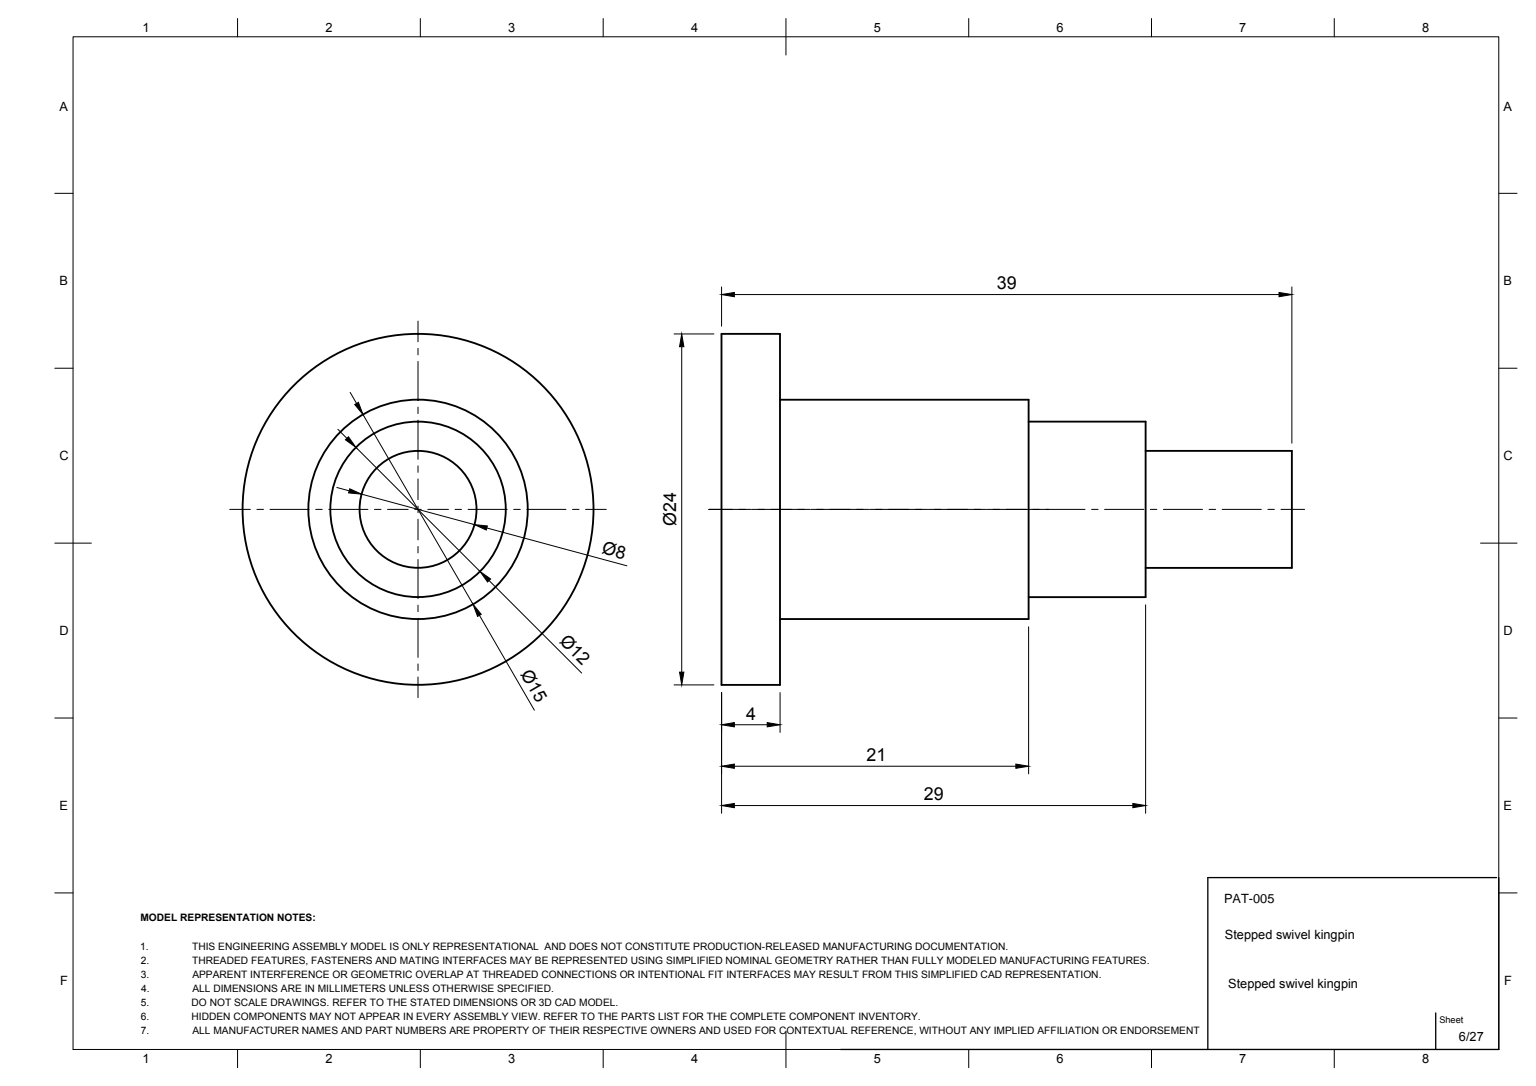
ISO-10303-21;
HEADER;
/* Generated by software containing ST-Developer
 * from STEP Tools, Inc. (www.steptools.com) 
 */

FILE_DESCRIPTION(
/* description */ ('Ball-race swivel caster'),
/* implementation_level */ '2;1');

FILE_NAME(
/* name */ 'Stepped swivel kingpin.step',
/* time_stamp */ '2026-10-29T16:15:51-07:00',
/* author */ (''),
/* organization */ (''),
/* preprocessor_version */ 'ST-DEVELOPER v20.2',
/* originating_system */ 'Autodesk Translation Framework v15.17.0.0',
/* authorisation */ '');

FILE_SCHEMA (('AUTOMOTIVE_DESIGN { 1 0 10303 214 3 1 1 }'));
ENDSEC;

DATA;
#10=MECHANICAL_DESIGN_GEOMETRIC_PRESENTATION_REPRESENTATION('',(#299),#7816);
#259=SHAPE_REPRESENTATION_RELATIONSHIP('SRR','None',#7904,#279);
#279=ADVANCED_BREP_SHAPE_REPRESENTATION('',(#335),#7793);
#299=STYLED_ITEM('',(#8097),#335);
#335=MANIFOLD_SOLID_BREP('Body1',#3705);
#379=FACE_BOUND('',#757,.T.);
#380=FACE_BOUND('',#761,.T.);
#381=FACE_BOUND('',#765,.T.);
#444=PLANE('',#3990);
#445=PLANE('',#3991);
#446=PLANE('',#3996);
#447=PLANE('',#3997);
#448=PLANE('',#4003);
#535=FACE_OUTER_BOUND('',#754,.T.);
#536=FACE_OUTER_BOUND('',#755,.T.);
#537=FACE_OUTER_BOUND('',#756,.T.);
#538=FACE_OUTER_BOUND('',#758,.T.);
#539=FACE_OUTER_BOUND('',#759,.T.);
#540=FACE_OUTER_BOUND('',#760,.T.);
#541=FACE_OUTER_BOUND('',#762,.T.);
#542=FACE_OUTER_BOUND('',#763,.T.);
#543=FACE_OUTER_BOUND('',#764,.T.);
#754=EDGE_LOOP('',(#2487,#2488,#2489,#2490));
#755=EDGE_LOOP('',(#2491));
#756=EDGE_LOOP('',(#2492));
#757=EDGE_LOOP('',(#2493));
#758=EDGE_LOOP('',(#2494,#2495,#2496,#2497));
#759=EDGE_LOOP('',(#2498));
#760=EDGE_LOOP('',(#2499));
#761=EDGE_LOOP('',(#2500));
#762=EDGE_LOOP('',(#2501,#2502,#2503,#2504));
#763=EDGE_LOOP('',(#2505,#2506,#2507,#2508));
#764=EDGE_LOOP('',(#2509));
#765=EDGE_LOOP('',(#2510));
#1028=LINE('',#5762,#1183);
#1029=LINE('',#5773,#1184);
#1030=LINE('',#5781,#1185);
#1031=LINE('',#5784,#1186);
#1183=VECTOR('',#4560,0.4);
#1184=VECTOR('',#4575,1.2);
#1185=VECTOR('',#4586,0.75);
#1186=VECTOR('',#4589,0.6);
#1331=CIRCLE('',#3988,0.4);
#1332=CIRCLE('',#3989,0.4);
#1333=CIRCLE('',#3992,1.2);
#1334=CIRCLE('',#3993,0.75);
#1335=CIRCLE('',#3995,1.2);
#1336=CIRCLE('',#3998,0.75);
#1337=CIRCLE('',#3999,0.6);
#1338=CIRCLE('',#4002,0.6);
#1603=VERTEX_POINT('',#5759);
#1604=VERTEX_POINT('',#5761);
#1605=VERTEX_POINT('',#5766);
#1606=VERTEX_POINT('',#5768);
#1607=VERTEX_POINT('',#5771);
#1608=VERTEX_POINT('',#5776);
#1609=VERTEX_POINT('',#5778);
#1610=VERTEX_POINT('',#5783);
#1963=EDGE_CURVE('',#1603,#1603,#1331,.T.);
#1964=EDGE_CURVE('',#1603,#1604,#1028,.T.);
#1965=EDGE_CURVE('',#1604,#1604,#1332,.T.);
#1966=EDGE_CURVE('',#1605,#1605,#1333,.T.);
#1967=EDGE_CURVE('',#1606,#1606,#1334,.T.);
#1968=EDGE_CURVE('',#1607,#1607,#1335,.T.);
#1969=EDGE_CURVE('',#1607,#1605,#1029,.T.);
#1970=EDGE_CURVE('',#1608,#1608,#1336,.T.);
#1971=EDGE_CURVE('',#1609,#1609,#1337,.T.);
#1972=EDGE_CURVE('',#1606,#1608,#1030,.T.);
#1973=EDGE_CURVE('',#1609,#1610,#1031,.T.);
#1974=EDGE_CURVE('',#1610,#1610,#1338,.T.);
#2487=ORIENTED_EDGE('',*,*,#1963,.F.);
#2488=ORIENTED_EDGE('',*,*,#1964,.T.);
#2489=ORIENTED_EDGE('',*,*,#1965,.T.);
#2490=ORIENTED_EDGE('',*,*,#1964,.F.);
#2491=ORIENTED_EDGE('',*,*,#1965,.F.);
#2492=ORIENTED_EDGE('',*,*,#1966,.F.);
#2493=ORIENTED_EDGE('',*,*,#1967,.T.);
#2494=ORIENTED_EDGE('',*,*,#1968,.F.);
#2495=ORIENTED_EDGE('',*,*,#1969,.T.);
#2496=ORIENTED_EDGE('',*,*,#1966,.T.);
#2497=ORIENTED_EDGE('',*,*,#1969,.F.);
#2498=ORIENTED_EDGE('',*,*,#1968,.T.);
#2499=ORIENTED_EDGE('',*,*,#1970,.F.);
#2500=ORIENTED_EDGE('',*,*,#1971,.T.);
#2501=ORIENTED_EDGE('',*,*,#1967,.F.);
#2502=ORIENTED_EDGE('',*,*,#1972,.T.);
#2503=ORIENTED_EDGE('',*,*,#1970,.T.);
#2504=ORIENTED_EDGE('',*,*,#1972,.F.);
#2505=ORIENTED_EDGE('',*,*,#1971,.F.);
#2506=ORIENTED_EDGE('',*,*,#1973,.T.);
#2507=ORIENTED_EDGE('',*,*,#1974,.T.);
#2508=ORIENTED_EDGE('',*,*,#1973,.F.);
#2509=ORIENTED_EDGE('',*,*,#1974,.F.);
#2510=ORIENTED_EDGE('',*,*,#1963,.T.);
#3432=CYLINDRICAL_SURFACE('',#3987,0.4);
#3433=CYLINDRICAL_SURFACE('',#3994,1.2);
#3434=CYLINDRICAL_SURFACE('',#4000,0.75);
#3435=CYLINDRICAL_SURFACE('',#4001,0.6);
#3506=ADVANCED_FACE('',(#535),#3432,.T.);
#3507=ADVANCED_FACE('',(#536),#444,.F.);
#3508=ADVANCED_FACE('',(#537,#379),#445,.F.);
#3509=ADVANCED_FACE('',(#538),#3433,.T.);
#3510=ADVANCED_FACE('',(#539),#446,.T.);
#3511=ADVANCED_FACE('',(#540,#380),#447,.F.);
#3512=ADVANCED_FACE('',(#541),#3434,.T.);
#3513=ADVANCED_FACE('',(#542),#3435,.T.);
#3514=ADVANCED_FACE('',(#543,#381),#448,.F.);
#3705=CLOSED_SHELL('',(#3506,#3507,#3508,#3509,#3510,#3511,#3512,#3513,
#3514));
#3986=AXIS2_PLACEMENT_3D('',#5757,#4554,#4555);
#3987=AXIS2_PLACEMENT_3D('',#5758,#4556,#4557);
#3988=AXIS2_PLACEMENT_3D('',#5760,#4558,#4559);
#3989=AXIS2_PLACEMENT_3D('',#5763,#4561,#4562);
#3990=AXIS2_PLACEMENT_3D('',#5764,#4563,#4564);
#3991=AXIS2_PLACEMENT_3D('',#5765,#4565,#4566);
#3992=AXIS2_PLACEMENT_3D('',#5767,#4567,#4568);
#3993=AXIS2_PLACEMENT_3D('',#5769,#4569,#4570);
#3994=AXIS2_PLACEMENT_3D('',#5770,#4571,#4572);
#3995=AXIS2_PLACEMENT_3D('',#5772,#4573,#4574);
#3996=AXIS2_PLACEMENT_3D('',#5774,#4576,#4577);
#3997=AXIS2_PLACEMENT_3D('',#5775,#4578,#4579);
#3998=AXIS2_PLACEMENT_3D('',#5777,#4580,#4581);
#3999=AXIS2_PLACEMENT_3D('',#5779,#4582,#4583);
#4000=AXIS2_PLACEMENT_3D('',#5780,#4584,#4585);
#4001=AXIS2_PLACEMENT_3D('',#5782,#4587,#4588);
#4002=AXIS2_PLACEMENT_3D('',#5785,#4590,#4591);
#4003=AXIS2_PLACEMENT_3D('',#5786,#4592,#4593);
#4554=DIRECTION('axis',(0.,0.,1.));
#4555=DIRECTION('refdir',(1.,0.,0.));
#4556=DIRECTION('center_axis',(0.,0.,1.));
#4557=DIRECTION('ref_axis',(1.,0.,0.));
#4558=DIRECTION('center_axis',(0.,0.,1.));
#4559=DIRECTION('ref_axis',(1.,0.,0.));
#4560=DIRECTION('',(0.,0.,-1.));
#4561=DIRECTION('center_axis',(0.,0.,1.));
#4562=DIRECTION('ref_axis',(1.,0.,0.));
#4563=DIRECTION('center_axis',(0.,0.,1.));
#4564=DIRECTION('ref_axis',(1.,0.,0.));
#4565=DIRECTION('center_axis',(0.,0.,1.));
#4566=DIRECTION('ref_axis',(1.,0.,0.));
#4567=DIRECTION('center_axis',(0.,0.,1.));
#4568=DIRECTION('ref_axis',(1.,0.,0.));
#4569=DIRECTION('center_axis',(0.,0.,1.));
#4570=DIRECTION('ref_axis',(1.,0.,0.));
#4571=DIRECTION('center_axis',(0.,0.,1.));
#4572=DIRECTION('ref_axis',(1.,0.,0.));
#4573=DIRECTION('center_axis',(0.,0.,1.));
#4574=DIRECTION('ref_axis',(1.,0.,0.));
#4575=DIRECTION('',(0.,0.,-1.));
#4576=DIRECTION('center_axis',(0.,0.,1.));
#4577=DIRECTION('ref_axis',(1.,0.,0.));
#4578=DIRECTION('center_axis',(0.,0.,1.));
#4579=DIRECTION('ref_axis',(1.,0.,0.));
#4580=DIRECTION('center_axis',(0.,0.,1.));
#4581=DIRECTION('ref_axis',(1.,0.,0.));
#4582=DIRECTION('center_axis',(0.,0.,1.));
#4583=DIRECTION('ref_axis',(1.,0.,0.));
#4584=DIRECTION('center_axis',(0.,0.,1.));
#4585=DIRECTION('ref_axis',(1.,0.,0.));
#4586=DIRECTION('',(0.,0.,-1.));
#4587=DIRECTION('center_axis',(0.,0.,1.));
#4588=DIRECTION('ref_axis',(1.,0.,0.));
#4589=DIRECTION('',(0.,0.,-1.));
#4590=DIRECTION('center_axis',(0.,0.,1.));
#4591=DIRECTION('ref_axis',(1.,0.,0.));
#4592=DIRECTION('center_axis',(0.,0.,1.));
#4593=DIRECTION('ref_axis',(1.,0.,0.));
#5757=CARTESIAN_POINT('',(0.,0.,0.));
#5758=CARTESIAN_POINT('Origin',(-2.,0.,7.5));
#5759=CARTESIAN_POINT('',(-2.4,-4.89858719658941E-17,8.5));
#5760=CARTESIAN_POINT('Origin',(-2.,0.,8.5));
#5761=CARTESIAN_POINT('',(-2.4,-4.89858719658941E-17,7.5));
#5762=CARTESIAN_POINT('',(-2.4,-4.89858719658941E-17,7.5));
#5763=CARTESIAN_POINT('Origin',(-2.,0.,7.5));
#5764=CARTESIAN_POINT('Origin',(-2.,0.,7.5));
#5765=CARTESIAN_POINT('Origin',(-2.,0.,11.));
#5766=CARTESIAN_POINT('',(-3.2,-1.46957615897682E-16,11.));
#5767=CARTESIAN_POINT('Origin',(-2.,0.,11.));
#5768=CARTESIAN_POINT('',(-2.75,-9.18485099360515E-17,11.));
#5769=CARTESIAN_POINT('Origin',(-2.,0.,11.));
#5770=CARTESIAN_POINT('Origin',(-2.,0.,11.));
#5771=CARTESIAN_POINT('',(-3.2,-1.46957615897682E-16,11.4));
#5772=CARTESIAN_POINT('Origin',(-2.,0.,11.4));
#5773=CARTESIAN_POINT('',(-3.2,-1.46957615897682E-16,11.));
#5774=CARTESIAN_POINT('Origin',(-2.,0.,11.4));
#5775=CARTESIAN_POINT('Origin',(-2.,0.,9.3));
#5776=CARTESIAN_POINT('',(-2.75,-9.18485099360515E-17,9.3));
#5777=CARTESIAN_POINT('Origin',(-2.,0.,9.3));
#5778=CARTESIAN_POINT('',(-2.6,-7.34788079488412E-17,9.3));
#5779=CARTESIAN_POINT('Origin',(-2.,0.,9.3));
#5780=CARTESIAN_POINT('Origin',(-2.,0.,9.3));
#5781=CARTESIAN_POINT('',(-2.75,-9.18485099360515E-17,9.3));
#5782=CARTESIAN_POINT('Origin',(-2.,0.,8.5));
#5783=CARTESIAN_POINT('',(-2.6,-7.34788079488412E-17,8.5));
#5784=CARTESIAN_POINT('',(-2.6,-7.34788079488412E-17,8.5));
#5785=CARTESIAN_POINT('Origin',(-2.,0.,8.5));
#5786=CARTESIAN_POINT('Origin',(-2.,0.,8.5));
#7766=UNCERTAINTY_MEASURE_WITH_UNIT(LENGTH_MEASURE(0.001),#7817,
'DISTANCE_ACCURACY_VALUE',
'Maximum model space distance between geometric entities at asserted c
onnectivities');
#7789=UNCERTAINTY_MEASURE_WITH_UNIT(LENGTH_MEASURE(0.001),#7817,
'DISTANCE_ACCURACY_VALUE',
'Maximum model space distance between geometric entities at asserted c
onnectivities');
#7793=(
GEOMETRIC_REPRESENTATION_CONTEXT(3)
GLOBAL_UNCERTAINTY_ASSIGNED_CONTEXT((#7766))
GLOBAL_UNIT_ASSIGNED_CONTEXT((#7817,#7819,#7820))
REPRESENTATION_CONTEXT('','3D')
);
#7816=(
GEOMETRIC_REPRESENTATION_CONTEXT(3)
GLOBAL_UNCERTAINTY_ASSIGNED_CONTEXT((#7789))
GLOBAL_UNIT_ASSIGNED_CONTEXT((#7817,#7819,#7820))
REPRESENTATION_CONTEXT('','3D')
);
#7817=(
LENGTH_UNIT()
NAMED_UNIT(*)
SI_UNIT(.CENTI.,.METRE.)
);
#7819=(
NAMED_UNIT(*)
PLANE_ANGLE_UNIT()
SI_UNIT($,.RADIAN.)
);
#7820=(
NAMED_UNIT(*)
SI_UNIT($,.STERADIAN.)
SOLID_ANGLE_UNIT()
);
#7824=SHAPE_DEFINITION_REPRESENTATION(#7850,#7904);
#7850=PRODUCT_DEFINITION_SHAPE('',$,#7931);
#7904=SHAPE_REPRESENTATION('',(#3986),#7793);
#7927=PRODUCT_DEFINITION_CONTEXT('part definition',#8007,'design');
#7931=PRODUCT_DEFINITION('Stepped swivel kingpin',
'Stepped swivel kingpin',#7957,#7927);
#7957=PRODUCT_DEFINITION_FORMATION('',$,#8012);
#8007=APPLICATION_CONTEXT(
'Core Data for Automotive Mechanical Design Process');
#8008=PRODUCT_CONTEXT('part definition',#8007,'mechanical');
#8012=PRODUCT('Stepped swivel kingpin','Stepped swivel kingpin',
'Stepped swivel kingpin',(#8008));
#8091=COLOUR_RGB('Grey',0.48,0.52,0.57);
#8092=FILL_AREA_STYLE_COLOUR('',#8091);
#8093=FILL_AREA_STYLE('',(#8092));
#8094=SURFACE_STYLE_FILL_AREA(#8093);
#8095=SURFACE_SIDE_STYLE('',(#8094));
#8096=SURFACE_STYLE_USAGE(.BOTH.,#8095);
#8097=PRESENTATION_STYLE_ASSIGNMENT((#8096));
ENDSEC;
END-ISO-10303-21;
